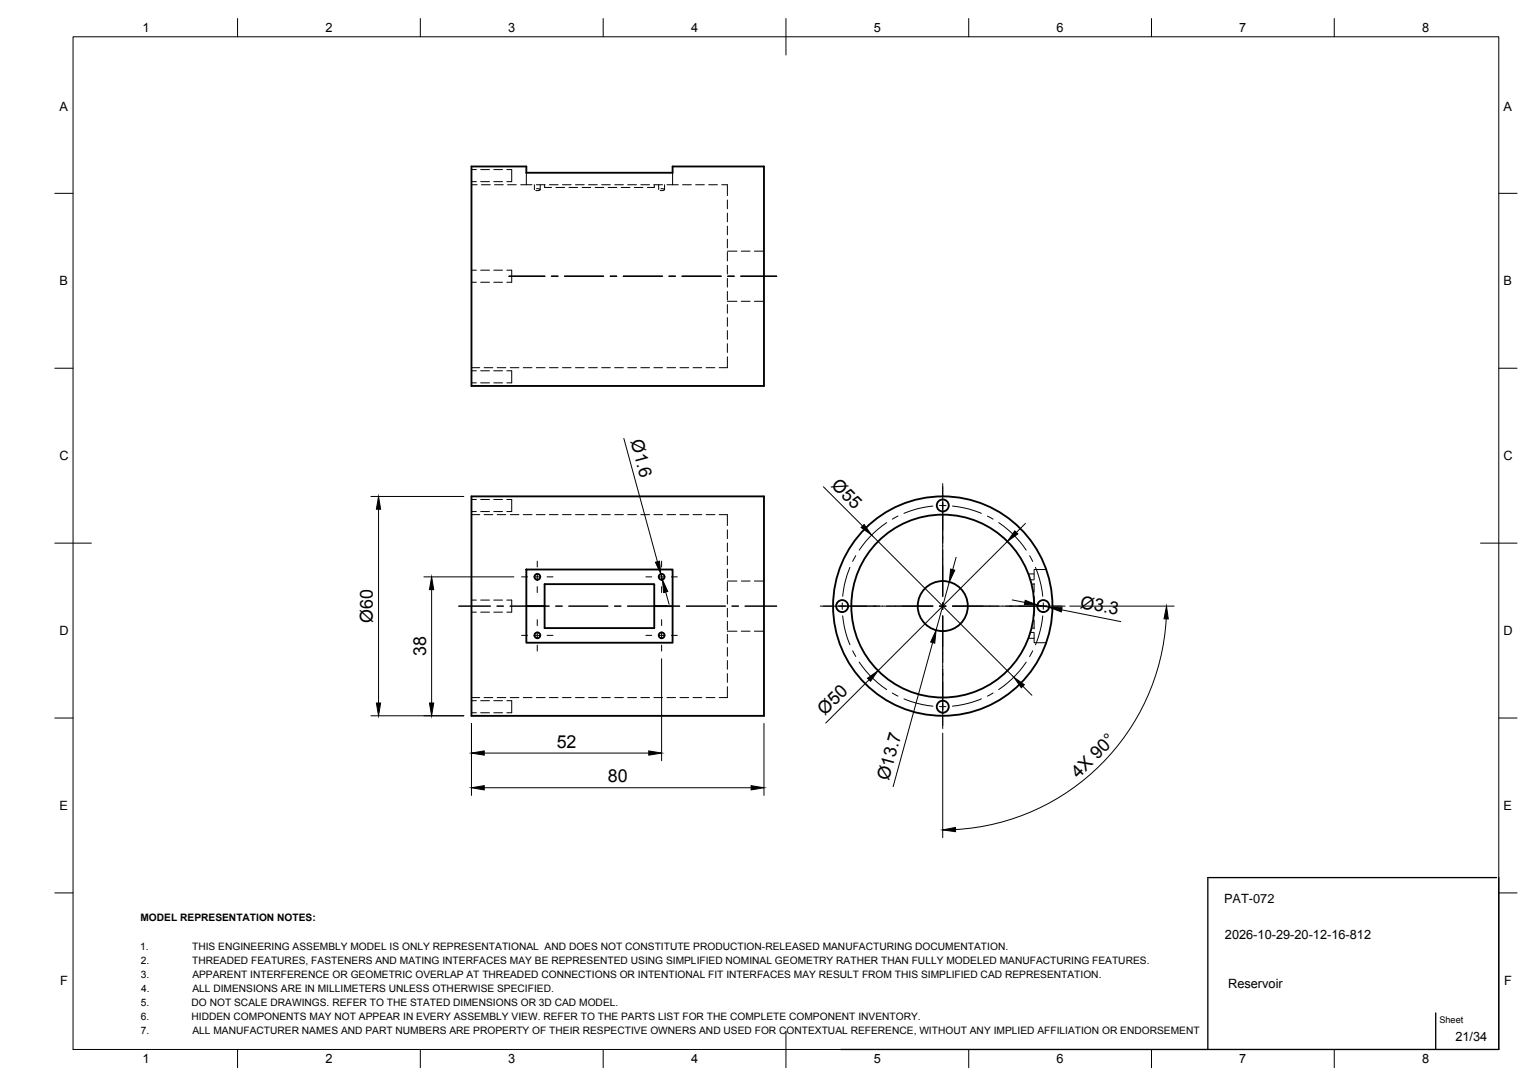
ISO-10303-21;
HEADER;
/* Generated by software containing ST-Developer
 * from STEP Tools, Inc. (www.steptools.com) 
 */

FILE_DESCRIPTION(
/* description */ ('PAT-072'),
/* implementation_level */ '2;1');

FILE_NAME(
/* name */ 'Reservoir.step',
/* time_stamp */ '2026-10-29T20:11:56-07:00',
/* author */ (''),
/* organization */ (''),
/* preprocessor_version */ 'ST-DEVELOPER v20.2',
/* originating_system */ 'Autodesk Translation Framework v15.17.0.0',
/* authorisation */ '');

FILE_SCHEMA (('AUTOMOTIVE_DESIGN { 1 0 10303 214 3 1 1 }'));
ENDSEC;

DATA;
#10=MECHANICAL_DESIGN_GEOMETRIC_PRESENTATION_REPRESENTATION('',(#350),#11432);
#249=B_SPLINE_CURVE_WITH_KNOTS('',3,(#10252,#10253,#10254,#10255,#10256,
#10257,#10258,#10259,#10260,#10261,#10262,#10263,#10264,#10265,#10266,#10267,
#10268,#10269,#10270,#10271,#10272,#10273,#10274,#10275,#10276,#10277,#10278,
#10279,#10280,#10281,#10282,#10283,#10284,#10285),.UNSPECIFIED.,.T.,.F.,
(4,2,2,2,2,2,2,2,2,2,2,2,2,2,2,2,4),(0.,0.0300404891334215,0.060080978266843,
0.0918437431465571,0.123606508026271,0.155653989866112,0.187701471705953,
0.217773943328409,0.247846414950866,0.277918886573323,0.30799135819578,
0.34003884003562,0.372086321875461,0.403849086755175,0.435611851634889,
0.465652340768311,0.495692829901732),.UNSPECIFIED.);
#250=B_SPLINE_CURVE_WITH_KNOTS('',3,(#10291,#10292,#10293,#10294,#10295,
#10296,#10297,#10298,#10299,#10300,#10301,#10302,#10303,#10304,#10305,#10306,
#10307,#10308,#10309,#10310,#10311,#10312,#10313,#10314,#10315,#10316,#10317,
#10318,#10319,#10320,#10321,#10322,#10323,#10324),.UNSPECIFIED.,.T.,.F.,
(4,2,2,2,2,2,2,2,2,2,2,2,2,2,2,2,4),(0.,0.0300724716224568,0.0601449432449135,
0.0921924250847542,0.124239906924595,0.156002671804309,0.187765436684023,
0.217805925817445,0.247846414950866,0.277886904084288,0.307927393217709,
0.339690158097423,0.371452922977137,0.403500404816978,0.435547886656819,
0.465620358279276,0.495692829901732),.UNSPECIFIED.);
#251=B_SPLINE_CURVE_WITH_KNOTS('',3,(#10330,#10331,#10332,#10333,#10334,
#10335,#10336,#10337,#10338,#10339,#10340,#10341,#10342,#10343,#10344,#10345,
#10346,#10347,#10348,#10349,#10350,#10351,#10352,#10353,#10354,#10355,#10356,
#10357,#10358,#10359,#10360,#10361,#10362,#10363),.UNSPECIFIED.,.T.,.F.,
(4,2,2,2,2,2,2,2,2,2,2,2,2,2,2,2,4),(0.,0.0300724716224568,0.0601449432449135,
0.0921924250847542,0.124239906924595,0.156002671804309,0.187765436684023,
0.217805925817445,0.247846414950866,0.277886904084288,0.307927393217709,
0.339690158097423,0.371452922977137,0.403500404816978,0.435547886656819,
0.465620358279276,0.495692829901732),.UNSPECIFIED.);
#252=B_SPLINE_CURVE_WITH_KNOTS('',3,(#10369,#10370,#10371,#10372,#10373,
#10374,#10375,#10376,#10377,#10378,#10379,#10380,#10381,#10382,#10383,#10384,
#10385,#10386,#10387,#10388,#10389,#10390,#10391,#10392,#10393,#10394,#10395,
#10396,#10397,#10398,#10399,#10400,#10401,#10402),.UNSPECIFIED.,.T.,.F.,
(4,2,2,2,2,2,2,2,2,2,2,2,2,2,2,2,4),(0.,0.0300404891334215,0.060080978266843,
0.0918437431465571,0.123606508026271,0.155653989866112,0.187701471705953,
0.217773943328409,0.247846414950866,0.277918886573323,0.30799135819578,
0.34003884003562,0.372086321875461,0.403849086755175,0.435611851634889,
0.465652340768311,0.495692829901732),.UNSPECIFIED.);
#278=SHAPE_REPRESENTATION_RELATIONSHIP('SRR','None',#11582,#314);
#314=ADVANCED_BREP_SHAPE_REPRESENTATION('',(#386),#11413);
#350=STYLED_ITEM('',(#11812),#386);
#386=MANIFOLD_SOLID_BREP('Body1',#6085);
#484=FACE_BOUND('',#1432,.T.);
#485=FACE_BOUND('',#1433,.T.);
#486=FACE_BOUND('',#1439,.T.);
#487=FACE_BOUND('',#1440,.T.);
#488=FACE_BOUND('',#1443,.T.);
#489=FACE_BOUND('',#1444,.T.);
#490=FACE_BOUND('',#1445,.T.);
#491=FACE_BOUND('',#1446,.T.);
#492=FACE_BOUND('',#1448,.T.);
#493=FACE_BOUND('',#1450,.T.);
#494=FACE_BOUND('',#1452,.T.);
#495=FACE_BOUND('',#1453,.T.);
#496=FACE_BOUND('',#1454,.T.);
#497=FACE_BOUND('',#1455,.T.);
#498=FACE_BOUND('',#1456,.T.);
#499=FACE_BOUND('',#1458,.T.);
#657=PLANE('',#6836);
#658=PLANE('',#6840);
#659=PLANE('',#6844);
#660=PLANE('',#6848);
#661=PLANE('',#6857);
#662=PLANE('',#6858);
#663=PLANE('',#6860);
#664=PLANE('',#6862);
#665=PLANE('',#6864);
#666=PLANE('',#6865);
#667=PLANE('',#6867);
#668=PLANE('',#6868);
#669=PLANE('',#6869);
#670=PLANE('',#6871);
#671=PLANE('',#6872);
#672=PLANE('',#6874);
#673=PLANE('',#6881);
#674=PLANE('',#6885);
#675=PLANE('',#6886);
#959=FACE_OUTER_BOUND('',#1413,.T.);
#960=FACE_OUTER_BOUND('',#1414,.T.);
#961=FACE_OUTER_BOUND('',#1415,.T.);
#962=FACE_OUTER_BOUND('',#1416,.T.);
#963=FACE_OUTER_BOUND('',#1417,.T.);
#964=FACE_OUTER_BOUND('',#1418,.T.);
#965=FACE_OUTER_BOUND('',#1419,.T.);
#966=FACE_OUTER_BOUND('',#1420,.T.);
#967=FACE_OUTER_BOUND('',#1421,.T.);
#968=FACE_OUTER_BOUND('',#1422,.T.);
#969=FACE_OUTER_BOUND('',#1423,.T.);
#970=FACE_OUTER_BOUND('',#1424,.T.);
#971=FACE_OUTER_BOUND('',#1425,.T.);
#972=FACE_OUTER_BOUND('',#1426,.T.);
#973=FACE_OUTER_BOUND('',#1427,.T.);
#974=FACE_OUTER_BOUND('',#1428,.T.);
#975=FACE_OUTER_BOUND('',#1429,.T.);
#976=FACE_OUTER_BOUND('',#1430,.T.);
#977=FACE_OUTER_BOUND('',#1431,.T.);
#978=FACE_OUTER_BOUND('',#1434,.T.);
#979=FACE_OUTER_BOUND('',#1435,.T.);
#980=FACE_OUTER_BOUND('',#1436,.T.);
#981=FACE_OUTER_BOUND('',#1437,.T.);
#982=FACE_OUTER_BOUND('',#1438,.T.);
#983=FACE_OUTER_BOUND('',#1441,.T.);
#984=FACE_OUTER_BOUND('',#1442,.T.);
#985=FACE_OUTER_BOUND('',#1447,.T.);
#986=FACE_OUTER_BOUND('',#1449,.T.);
#987=FACE_OUTER_BOUND('',#1451,.T.);
#988=FACE_OUTER_BOUND('',#1457,.T.);
#1413=EDGE_LOOP('',(#4678,#4679,#4680,#4681));
#1414=EDGE_LOOP('',(#4682));
#1415=EDGE_LOOP('',(#4683,#4684,#4685,#4686));
#1416=EDGE_LOOP('',(#4687));
#1417=EDGE_LOOP('',(#4688,#4689,#4690,#4691));
#1418=EDGE_LOOP('',(#4692));
#1419=EDGE_LOOP('',(#4693,#4694,#4695,#4696));
#1420=EDGE_LOOP('',(#4697));
#1421=EDGE_LOOP('',(#4698,#4699,#4700,#4701));
#1422=EDGE_LOOP('',(#4702,#4703,#4704,#4705));
#1423=EDGE_LOOP('',(#4706,#4707,#4708,#4709));
#1424=EDGE_LOOP('',(#4710,#4711,#4712,#4713));
#1425=EDGE_LOOP('',(#4714,#4715,#4716,#4717));
#1426=EDGE_LOOP('',(#4718,#4719,#4720));
#1427=EDGE_LOOP('',(#4721,#4722,#4723));
#1428=EDGE_LOOP('',(#4724,#4725,#4726));
#1429=EDGE_LOOP('',(#4727,#4728,#4729,#4730));
#1430=EDGE_LOOP('',(#4731,#4732,#4733));
#1431=EDGE_LOOP('',(#4734,#4735,#4736,#4737,#4738,#4739,#4740,#4741));
#1432=EDGE_LOOP('',(#4742));
#1433=EDGE_LOOP('',(#4743));
#1434=EDGE_LOOP('',(#4744,#4745,#4746,#4747));
#1435=EDGE_LOOP('',(#4748,#4749,#4750,#4751,#4752));
#1436=EDGE_LOOP('',(#4753,#4754,#4755,#4756));
#1437=EDGE_LOOP('',(#4757,#4758,#4759,#4760,#4761));
#1438=EDGE_LOOP('',(#4762,#4763,#4764,#4765,#4766,#4767,#4768,#4769));
#1439=EDGE_LOOP('',(#4770));
#1440=EDGE_LOOP('',(#4771));
#1441=EDGE_LOOP('',(#4772,#4773,#4774,#4775));
#1442=EDGE_LOOP('',(#4776,#4777,#4778,#4779,#4780,#4781,#4782,#4783,#4784,
#4785,#4786,#4787,#4788,#4789,#4790,#4791));
#1443=EDGE_LOOP('',(#4792));
#1444=EDGE_LOOP('',(#4793));
#1445=EDGE_LOOP('',(#4794));
#1446=EDGE_LOOP('',(#4795));
#1447=EDGE_LOOP('',(#4796));
#1448=EDGE_LOOP('',(#4797));
#1449=EDGE_LOOP('',(#4798,#4799,#4800,#4801));
#1450=EDGE_LOOP('',(#4802,#4803,#4804,#4805));
#1451=EDGE_LOOP('',(#4806));
#1452=EDGE_LOOP('',(#4807));
#1453=EDGE_LOOP('',(#4808));
#1454=EDGE_LOOP('',(#4809));
#1455=EDGE_LOOP('',(#4810));
#1456=EDGE_LOOP('',(#4811));
#1457=EDGE_LOOP('',(#4812));
#1458=EDGE_LOOP('',(#4813));
#1840=LINE('',#10223,#2259);
#1841=LINE('',#10230,#2260);
#1842=LINE('',#10237,#2261);
#1843=LINE('',#10244,#2262);
#1844=LINE('',#10251,#2263);
#1845=LINE('',#10290,#2264);
#1846=LINE('',#10329,#2265);
#1847=LINE('',#10368,#2266);
#1848=LINE('',#10406,#2267);
#1849=LINE('',#10408,#2268);
#1850=LINE('',#10410,#2269);
#1851=LINE('',#10411,#2270);
#1852=LINE('',#10417,#2271);
#1853=LINE('',#10418,#2272);
#1854=LINE('',#10424,#2273);
#1855=LINE('',#10425,#2274);
#1856=LINE('',#10428,#2275);
#1857=LINE('',#10430,#2276);
#1858=LINE('',#10431,#2277);
#1859=LINE('',#10434,#2278);
#1860=LINE('',#10437,#2279);
#1861=LINE('',#10439,#2280);
#1862=LINE('',#10441,#2281);
#1863=LINE('',#10443,#2282);
#1864=LINE('',#10444,#2283);
#1865=LINE('',#10448,#2284);
#1866=LINE('',#10449,#2285);
#1867=LINE('',#10450,#2286);
#1868=LINE('',#10455,#2287);
#1869=LINE('',#10456,#2288);
#1870=LINE('',#10459,#2289);
#1871=LINE('',#10461,#2290);
#1872=LINE('',#10462,#2291);
#1873=LINE('',#10465,#2292);
#1874=LINE('',#10467,#2293);
#1875=LINE('',#10468,#2294);
#1876=LINE('',#10473,#2295);
#1877=LINE('',#10478,#2296);
#1878=LINE('',#10480,#2297);
#1879=LINE('',#10487,#2298);
#2259=VECTOR('',#8057,0.165);
#2260=VECTOR('',#8066,0.165);
#2261=VECTOR('',#8075,0.165);
#2262=VECTOR('',#8084,0.165);
#2263=VECTOR('',#8093,0.08);
#2264=VECTOR('',#8098,0.08);
#2265=VECTOR('',#8103,0.08);
#2266=VECTOR('',#8108,0.08);
#2267=VECTOR('',#8111,1.);
#2268=VECTOR('',#8112,1.);
#2269=VECTOR('',#8113,1.);
#2270=VECTOR('',#8114,1.);
#2271=VECTOR('',#8119,1.);
#2272=VECTOR('',#8120,1.);
#2273=VECTOR('',#8125,1.);
#2274=VECTOR('',#8126,1.);
#2275=VECTOR('',#8131,1.);
#2276=VECTOR('',#8134,1.);
#2277=VECTOR('',#8135,1.);
#2278=VECTOR('',#8140,1.);
#2279=VECTOR('',#8143,1.);
#2280=VECTOR('',#8144,1.);
#2281=VECTOR('',#8145,1.);
#2282=VECTOR('',#8146,1.);
#2283=VECTOR('',#8147,1.);
#2284=VECTOR('',#8150,1.);
#2285=VECTOR('',#8151,1.);
#2286=VECTOR('',#8152,1.);
#2287=VECTOR('',#8157,1.);
#2288=VECTOR('',#8158,1.);
#2289=VECTOR('',#8161,1.);
#2290=VECTOR('',#8162,1.);
#2291=VECTOR('',#8163,1.);
#2292=VECTOR('',#8168,1.);
#2293=VECTOR('',#8171,1.);
#2294=VECTOR('',#8172,1.);
#2295=VECTOR('',#8177,0.685);
#2296=VECTOR('',#8184,2.5);
#2297=VECTOR('',#8185,2.5);
#2298=VECTOR('',#8194,3.);
#2687=CIRCLE('',#6834,0.165);
#2688=CIRCLE('',#6835,0.165);
#2689=CIRCLE('',#6838,0.165);
#2690=CIRCLE('',#6839,0.165);
#2691=CIRCLE('',#6842,0.165);
#2692=CIRCLE('',#6843,0.165);
#2693=CIRCLE('',#6846,0.165);
#2694=CIRCLE('',#6847,0.165);
#2695=CIRCLE('',#6850,0.08);
#2696=CIRCLE('',#6852,0.08);
#2697=CIRCLE('',#6854,0.08);
#2698=CIRCLE('',#6856,0.08);
#2699=CIRCLE('',#6859,2.5);
#2700=CIRCLE('',#6861,2.5);
#2701=CIRCLE('',#6863,2.5);
#2702=CIRCLE('',#6866,2.5);
#2703=CIRCLE('',#6870,3.);
#2704=CIRCLE('',#6873,3.);
#2705=CIRCLE('',#6876,0.685);
#2706=CIRCLE('',#6877,0.685);
#2707=CIRCLE('',#6879,2.5);
#2708=CIRCLE('',#6880,2.5);
#2709=CIRCLE('',#6883,3.);
#2710=CIRCLE('',#6884,3.);
#3036=VERTEX_POINT('',#10220);
#3037=VERTEX_POINT('',#10222);
#3038=VERTEX_POINT('',#10227);
#3039=VERTEX_POINT('',#10229);
#3040=VERTEX_POINT('',#10234);
#3041=VERTEX_POINT('',#10236);
#3042=VERTEX_POINT('',#10241);
#3043=VERTEX_POINT('',#10243);
#3044=VERTEX_POINT('',#10248);
#3045=VERTEX_POINT('',#10250);
#3046=VERTEX_POINT('',#10287);
#3047=VERTEX_POINT('',#10289);
#3048=VERTEX_POINT('',#10326);
#3049=VERTEX_POINT('',#10328);
#3050=VERTEX_POINT('',#10365);
#3051=VERTEX_POINT('',#10367);
#3052=VERTEX_POINT('',#10404);
#3053=VERTEX_POINT('',#10405);
#3054=VERTEX_POINT('',#10407);
#3055=VERTEX_POINT('',#10409);
#3056=VERTEX_POINT('',#10413);
#3057=VERTEX_POINT('',#10414);
#3058=VERTEX_POINT('',#10416);
#3059=VERTEX_POINT('',#10420);
#3060=VERTEX_POINT('',#10421);
#3061=VERTEX_POINT('',#10423);
#3062=VERTEX_POINT('',#10436);
#3063=VERTEX_POINT('',#10438);
#3064=VERTEX_POINT('',#10440);
#3065=VERTEX_POINT('',#10442);
#3066=VERTEX_POINT('',#10446);
#3067=VERTEX_POINT('',#10447);
#3068=VERTEX_POINT('',#10452);
#3069=VERTEX_POINT('',#10454);
#3070=VERTEX_POINT('',#10458);
#3071=VERTEX_POINT('',#10460);
#3072=VERTEX_POINT('',#10470);
#3073=VERTEX_POINT('',#10472);
#3074=VERTEX_POINT('',#10476);
#3075=VERTEX_POINT('',#10479);
#3076=VERTEX_POINT('',#10484);
#3077=VERTEX_POINT('',#10486);
#3628=EDGE_CURVE('',#3036,#3036,#2687,.T.);
#3629=EDGE_CURVE('',#3036,#3037,#1840,.T.);
#3630=EDGE_CURVE('',#3037,#3037,#2688,.T.);
#3631=EDGE_CURVE('',#3038,#3038,#2689,.T.);
#3632=EDGE_CURVE('',#3038,#3039,#1841,.T.);
#3633=EDGE_CURVE('',#3039,#3039,#2690,.T.);
#3634=EDGE_CURVE('',#3040,#3040,#2691,.T.);
#3635=EDGE_CURVE('',#3040,#3041,#1842,.T.);
#3636=EDGE_CURVE('',#3041,#3041,#2692,.T.);
#3637=EDGE_CURVE('',#3042,#3042,#2693,.T.);
#3638=EDGE_CURVE('',#3042,#3043,#1843,.T.);
#3639=EDGE_CURVE('',#3043,#3043,#2694,.T.);
#3640=EDGE_CURVE('',#3044,#3044,#2695,.T.);
#3641=EDGE_CURVE('',#3044,#3045,#1844,.T.);
#3642=EDGE_CURVE('',#3045,#3045,#249,.T.);
#3643=EDGE_CURVE('',#3046,#3046,#2696,.T.);
#3644=EDGE_CURVE('',#3046,#3047,#1845,.T.);
#3645=EDGE_CURVE('',#3047,#3047,#250,.T.);
#3646=EDGE_CURVE('',#3048,#3048,#2697,.T.);
#3647=EDGE_CURVE('',#3048,#3049,#1846,.T.);
#3648=EDGE_CURVE('',#3049,#3049,#251,.T.);
#3649=EDGE_CURVE('',#3050,#3050,#2698,.T.);
#3650=EDGE_CURVE('',#3050,#3051,#1847,.T.);
#3651=EDGE_CURVE('',#3051,#3051,#252,.T.);
#3652=EDGE_CURVE('',#3052,#3053,#1848,.T.);
#3653=EDGE_CURVE('',#3054,#3052,#1849,.T.);
#3654=EDGE_CURVE('',#3055,#3054,#1850,.T.);
#3655=EDGE_CURVE('',#3055,#3053,#1851,.T.);
#3656=EDGE_CURVE('',#3056,#3057,#2699,.T.);
#3657=EDGE_CURVE('',#3058,#3056,#1852,.T.);
#3658=EDGE_CURVE('',#3057,#3058,#1853,.T.);
#3659=EDGE_CURVE('',#3059,#3060,#2700,.T.);
#3660=EDGE_CURVE('',#3061,#3059,#1854,.T.);
#3661=EDGE_CURVE('',#3061,#3060,#1855,.T.);
#3662=EDGE_CURVE('',#3053,#3059,#2701,.T.);
#3663=EDGE_CURVE('',#3059,#3055,#1856,.T.);
#3664=EDGE_CURVE('',#3060,#3056,#1857,.T.);
#3665=EDGE_CURVE('',#3058,#3061,#1858,.T.);
#3666=EDGE_CURVE('',#3057,#3052,#2702,.T.);
#3667=EDGE_CURVE('',#3054,#3057,#1859,.T.);
#3668=EDGE_CURVE('',#3059,#3062,#1860,.T.);
#3669=EDGE_CURVE('',#3063,#3062,#1861,.T.);
#3670=EDGE_CURVE('',#3064,#3063,#1862,.T.);
#3671=EDGE_CURVE('',#3065,#3064,#1863,.T.);
#3672=EDGE_CURVE('',#3065,#3057,#1864,.T.);
#3673=EDGE_CURVE('',#3066,#3067,#1865,.T.);
#3674=EDGE_CURVE('',#3066,#3064,#1866,.T.);
#3675=EDGE_CURVE('',#3067,#3063,#1867,.T.);
#3676=EDGE_CURVE('',#3067,#3068,#2703,.T.);
#3677=EDGE_CURVE('',#3062,#3069,#1868,.T.);
#3678=EDGE_CURVE('',#3068,#3069,#1869,.T.);
#3679=EDGE_CURVE('',#3068,#3070,#1870,.T.);
#3680=EDGE_CURVE('',#3069,#3071,#1871,.T.);
#3681=EDGE_CURVE('',#3070,#3071,#1872,.T.);
#3682=EDGE_CURVE('',#3070,#3066,#2704,.T.);
#3683=EDGE_CURVE('',#3071,#3065,#1873,.T.);
#3684=EDGE_CURVE('',#3065,#3057,#1874,.T.);
#3685=EDGE_CURVE('',#3059,#3062,#1875,.T.);
#3686=EDGE_CURVE('',#3072,#3072,#2705,.T.);
#3687=EDGE_CURVE('',#3072,#3073,#1876,.T.);
#3688=EDGE_CURVE('',#3073,#3073,#2706,.T.);
#3689=EDGE_CURVE('',#3074,#3074,#2707,.T.);
#3690=EDGE_CURVE('',#3074,#3062,#1877,.T.);
#3691=EDGE_CURVE('',#3065,#3075,#1878,.T.);
#3692=EDGE_CURVE('',#3075,#3075,#2708,.T.);
#3693=EDGE_CURVE('',#3076,#3076,#2709,.T.);
#3694=EDGE_CURVE('',#3076,#3077,#1879,.T.);
#3695=EDGE_CURVE('',#3077,#3077,#2710,.T.);
#4678=ORIENTED_EDGE('',*,*,#3628,.F.);
#4679=ORIENTED_EDGE('',*,*,#3629,.T.);
#4680=ORIENTED_EDGE('',*,*,#3630,.F.);
#4681=ORIENTED_EDGE('',*,*,#3629,.F.);
#4682=ORIENTED_EDGE('',*,*,#3628,.T.);
#4683=ORIENTED_EDGE('',*,*,#3631,.F.);
#4684=ORIENTED_EDGE('',*,*,#3632,.T.);
#4685=ORIENTED_EDGE('',*,*,#3633,.F.);
#4686=ORIENTED_EDGE('',*,*,#3632,.F.);
#4687=ORIENTED_EDGE('',*,*,#3631,.T.);
#4688=ORIENTED_EDGE('',*,*,#3634,.F.);
#4689=ORIENTED_EDGE('',*,*,#3635,.T.);
#4690=ORIENTED_EDGE('',*,*,#3636,.F.);
#4691=ORIENTED_EDGE('',*,*,#3635,.F.);
#4692=ORIENTED_EDGE('',*,*,#3634,.T.);
#4693=ORIENTED_EDGE('',*,*,#3637,.F.);
#4694=ORIENTED_EDGE('',*,*,#3638,.T.);
#4695=ORIENTED_EDGE('',*,*,#3639,.F.);
#4696=ORIENTED_EDGE('',*,*,#3638,.F.);
#4697=ORIENTED_EDGE('',*,*,#3637,.T.);
#4698=ORIENTED_EDGE('',*,*,#3640,.F.);
#4699=ORIENTED_EDGE('',*,*,#3641,.T.);
#4700=ORIENTED_EDGE('',*,*,#3642,.F.);
#4701=ORIENTED_EDGE('',*,*,#3641,.F.);
#4702=ORIENTED_EDGE('',*,*,#3643,.F.);
#4703=ORIENTED_EDGE('',*,*,#3644,.T.);
#4704=ORIENTED_EDGE('',*,*,#3645,.F.);
#4705=ORIENTED_EDGE('',*,*,#3644,.F.);
#4706=ORIENTED_EDGE('',*,*,#3646,.F.);
#4707=ORIENTED_EDGE('',*,*,#3647,.T.);
#4708=ORIENTED_EDGE('',*,*,#3648,.F.);
#4709=ORIENTED_EDGE('',*,*,#3647,.F.);
#4710=ORIENTED_EDGE('',*,*,#3649,.F.);
#4711=ORIENTED_EDGE('',*,*,#3650,.T.);
#4712=ORIENTED_EDGE('',*,*,#3651,.F.);
#4713=ORIENTED_EDGE('',*,*,#3650,.F.);
#4714=ORIENTED_EDGE('',*,*,#3652,.F.);
#4715=ORIENTED_EDGE('',*,*,#3653,.F.);
#4716=ORIENTED_EDGE('',*,*,#3654,.F.);
#4717=ORIENTED_EDGE('',*,*,#3655,.T.);
#4718=ORIENTED_EDGE('',*,*,#3656,.F.);
#4719=ORIENTED_EDGE('',*,*,#3657,.F.);
#4720=ORIENTED_EDGE('',*,*,#3658,.F.);
#4721=ORIENTED_EDGE('',*,*,#3659,.F.);
#4722=ORIENTED_EDGE('',*,*,#3660,.F.);
#4723=ORIENTED_EDGE('',*,*,#3661,.T.);
#4724=ORIENTED_EDGE('',*,*,#3662,.F.);
#4725=ORIENTED_EDGE('',*,*,#3655,.F.);
#4726=ORIENTED_EDGE('',*,*,#3663,.F.);
#4727=ORIENTED_EDGE('',*,*,#3664,.F.);
#4728=ORIENTED_EDGE('',*,*,#3661,.F.);
#4729=ORIENTED_EDGE('',*,*,#3665,.F.);
#4730=ORIENTED_EDGE('',*,*,#3657,.T.);
#4731=ORIENTED_EDGE('',*,*,#3666,.F.);
#4732=ORIENTED_EDGE('',*,*,#3667,.F.);
#4733=ORIENTED_EDGE('',*,*,#3653,.T.);
#4734=ORIENTED_EDGE('',*,*,#3658,.T.);
#4735=ORIENTED_EDGE('',*,*,#3665,.T.);
#4736=ORIENTED_EDGE('',*,*,#3660,.T.);
#4737=ORIENTED_EDGE('',*,*,#3668,.T.);
#4738=ORIENTED_EDGE('',*,*,#3669,.F.);
#4739=ORIENTED_EDGE('',*,*,#3670,.F.);
#4740=ORIENTED_EDGE('',*,*,#3671,.F.);
#4741=ORIENTED_EDGE('',*,*,#3672,.T.);
#4742=ORIENTED_EDGE('',*,*,#3640,.T.);
#4743=ORIENTED_EDGE('',*,*,#3649,.T.);
#4744=ORIENTED_EDGE('',*,*,#3673,.F.);
#4745=ORIENTED_EDGE('',*,*,#3674,.T.);
#4746=ORIENTED_EDGE('',*,*,#3670,.T.);
#4747=ORIENTED_EDGE('',*,*,#3675,.F.);
#4748=ORIENTED_EDGE('',*,*,#3676,.F.);
#4749=ORIENTED_EDGE('',*,*,#3675,.T.);
#4750=ORIENTED_EDGE('',*,*,#3669,.T.);
#4751=ORIENTED_EDGE('',*,*,#3677,.T.);
#4752=ORIENTED_EDGE('',*,*,#3678,.F.);
#4753=ORIENTED_EDGE('',*,*,#3679,.F.);
#4754=ORIENTED_EDGE('',*,*,#3678,.T.);
#4755=ORIENTED_EDGE('',*,*,#3680,.T.);
#4756=ORIENTED_EDGE('',*,*,#3681,.F.);
#4757=ORIENTED_EDGE('',*,*,#3682,.F.);
#4758=ORIENTED_EDGE('',*,*,#3681,.T.);
#4759=ORIENTED_EDGE('',*,*,#3683,.T.);
#4760=ORIENTED_EDGE('',*,*,#3671,.T.);
#4761=ORIENTED_EDGE('',*,*,#3674,.F.);
#4762=ORIENTED_EDGE('',*,*,#3667,.T.);
#4763=ORIENTED_EDGE('',*,*,#3684,.F.);
#4764=ORIENTED_EDGE('',*,*,#3683,.F.);
#4765=ORIENTED_EDGE('',*,*,#3680,.F.);
#4766=ORIENTED_EDGE('',*,*,#3677,.F.);
#4767=ORIENTED_EDGE('',*,*,#3685,.F.);
#4768=ORIENTED_EDGE('',*,*,#3663,.T.);
#4769=ORIENTED_EDGE('',*,*,#3654,.T.);
#4770=ORIENTED_EDGE('',*,*,#3643,.T.);
#4771=ORIENTED_EDGE('',*,*,#3646,.T.);
#4772=ORIENTED_EDGE('',*,*,#3686,.F.);
#4773=ORIENTED_EDGE('',*,*,#3687,.T.);
#4774=ORIENTED_EDGE('',*,*,#3688,.F.);
#4775=ORIENTED_EDGE('',*,*,#3687,.F.);
#4776=ORIENTED_EDGE('',*,*,#3689,.F.);
#4777=ORIENTED_EDGE('',*,*,#3690,.T.);
#4778=ORIENTED_EDGE('',*,*,#3668,.F.);
#4779=ORIENTED_EDGE('',*,*,#3659,.T.);
#4780=ORIENTED_EDGE('',*,*,#3664,.T.);
#4781=ORIENTED_EDGE('',*,*,#3656,.T.);
#4782=ORIENTED_EDGE('',*,*,#3672,.F.);
#4783=ORIENTED_EDGE('',*,*,#3691,.T.);
#4784=ORIENTED_EDGE('',*,*,#3692,.F.);
#4785=ORIENTED_EDGE('',*,*,#3691,.F.);
#4786=ORIENTED_EDGE('',*,*,#3684,.T.);
#4787=ORIENTED_EDGE('',*,*,#3666,.T.);
#4788=ORIENTED_EDGE('',*,*,#3652,.T.);
#4789=ORIENTED_EDGE('',*,*,#3662,.T.);
#4790=ORIENTED_EDGE('',*,*,#3685,.T.);
#4791=ORIENTED_EDGE('',*,*,#3690,.F.);
#4792=ORIENTED_EDGE('',*,*,#3642,.T.);
#4793=ORIENTED_EDGE('',*,*,#3645,.T.);
#4794=ORIENTED_EDGE('',*,*,#3648,.T.);
#4795=ORIENTED_EDGE('',*,*,#3651,.T.);
#4796=ORIENTED_EDGE('',*,*,#3689,.T.);
#4797=ORIENTED_EDGE('',*,*,#3688,.T.);
#4798=ORIENTED_EDGE('',*,*,#3693,.F.);
#4799=ORIENTED_EDGE('',*,*,#3694,.T.);
#4800=ORIENTED_EDGE('',*,*,#3695,.T.);
#4801=ORIENTED_EDGE('',*,*,#3694,.F.);
#4802=ORIENTED_EDGE('',*,*,#3679,.T.);
#4803=ORIENTED_EDGE('',*,*,#3682,.T.);
#4804=ORIENTED_EDGE('',*,*,#3673,.T.);
#4805=ORIENTED_EDGE('',*,*,#3676,.T.);
#4806=ORIENTED_EDGE('',*,*,#3693,.T.);
#4807=ORIENTED_EDGE('',*,*,#3692,.T.);
#4808=ORIENTED_EDGE('',*,*,#3639,.T.);
#4809=ORIENTED_EDGE('',*,*,#3636,.T.);
#4810=ORIENTED_EDGE('',*,*,#3633,.T.);
#4811=ORIENTED_EDGE('',*,*,#3630,.T.);
#4812=ORIENTED_EDGE('',*,*,#3695,.F.);
#4813=ORIENTED_EDGE('',*,*,#3686,.T.);
#5634=CYLINDRICAL_SURFACE('',#6833,0.165);
#5635=CYLINDRICAL_SURFACE('',#6837,0.165);
#5636=CYLINDRICAL_SURFACE('',#6841,0.165);
#5637=CYLINDRICAL_SURFACE('',#6845,0.165);
#5638=CYLINDRICAL_SURFACE('',#6849,0.08);
#5639=CYLINDRICAL_SURFACE('',#6851,0.08);
#5640=CYLINDRICAL_SURFACE('',#6853,0.08);
#5641=CYLINDRICAL_SURFACE('',#6855,0.08);
#5642=CYLINDRICAL_SURFACE('',#6875,0.685);
#5643=CYLINDRICAL_SURFACE('',#6878,2.5);
#5644=CYLINDRICAL_SURFACE('',#6882,3.);
#5858=ADVANCED_FACE('',(#959),#5634,.F.);
#5859=ADVANCED_FACE('',(#960),#657,.T.);
#5860=ADVANCED_FACE('',(#961),#5635,.F.);
#5861=ADVANCED_FACE('',(#962),#658,.T.);
#5862=ADVANCED_FACE('',(#963),#5636,.F.);
#5863=ADVANCED_FACE('',(#964),#659,.T.);
#5864=ADVANCED_FACE('',(#965),#5637,.F.);
#5865=ADVANCED_FACE('',(#966),#660,.T.);
#5866=ADVANCED_FACE('',(#967),#5638,.F.);
#5867=ADVANCED_FACE('',(#968),#5639,.F.);
#5868=ADVANCED_FACE('',(#969),#5640,.F.);
#5869=ADVANCED_FACE('',(#970),#5641,.F.);
#5870=ADVANCED_FACE('',(#971),#661,.F.);
#5871=ADVANCED_FACE('',(#972),#662,.F.);
#5872=ADVANCED_FACE('',(#973),#663,.F.);
#5873=ADVANCED_FACE('',(#974),#664,.F.);
#5874=ADVANCED_FACE('',(#975),#665,.F.);
#5875=ADVANCED_FACE('',(#976),#666,.F.);
#5876=ADVANCED_FACE('',(#977,#484,#485),#667,.F.);
#5877=ADVANCED_FACE('',(#978),#668,.F.);
#5878=ADVANCED_FACE('',(#979),#669,.F.);
#5879=ADVANCED_FACE('',(#980),#670,.F.);
#5880=ADVANCED_FACE('',(#981),#671,.F.);
#5881=ADVANCED_FACE('',(#982,#486,#487),#672,.F.);
#5882=ADVANCED_FACE('',(#983),#5642,.F.);
#5883=ADVANCED_FACE('',(#984,#488,#489,#490,#491),#5643,.F.);
#5884=ADVANCED_FACE('',(#985,#492),#673,.T.);
#5885=ADVANCED_FACE('',(#986,#493),#5644,.T.);
#5886=ADVANCED_FACE('',(#987,#494,#495,#496,#497,#498),#674,.T.);
#5887=ADVANCED_FACE('',(#988,#499),#675,.F.);
#6085=CLOSED_SHELL('',(#5858,#5859,#5860,#5861,#5862,#5863,#5864,#5865,
#5866,#5867,#5868,#5869,#5870,#5871,#5872,#5873,#5874,#5875,#5876,#5877,
#5878,#5879,#5880,#5881,#5882,#5883,#5884,#5885,#5886,#5887));
#6832=AXIS2_PLACEMENT_3D('',#10218,#8051,#8052);
#6833=AXIS2_PLACEMENT_3D('',#10219,#8053,#8054);
#6834=AXIS2_PLACEMENT_3D('',#10221,#8055,#8056);
#6835=AXIS2_PLACEMENT_3D('',#10224,#8058,#8059);
#6836=AXIS2_PLACEMENT_3D('',#10225,#8060,#8061);
#6837=AXIS2_PLACEMENT_3D('',#10226,#8062,#8063);
#6838=AXIS2_PLACEMENT_3D('',#10228,#8064,#8065);
#6839=AXIS2_PLACEMENT_3D('',#10231,#8067,#8068);
#6840=AXIS2_PLACEMENT_3D('',#10232,#8069,#8070);
#6841=AXIS2_PLACEMENT_3D('',#10233,#8071,#8072);
#6842=AXIS2_PLACEMENT_3D('',#10235,#8073,#8074);
#6843=AXIS2_PLACEMENT_3D('',#10238,#8076,#8077);
#6844=AXIS2_PLACEMENT_3D('',#10239,#8078,#8079);
#6845=AXIS2_PLACEMENT_3D('',#10240,#8080,#8081);
#6846=AXIS2_PLACEMENT_3D('',#10242,#8082,#8083);
#6847=AXIS2_PLACEMENT_3D('',#10245,#8085,#8086);
#6848=AXIS2_PLACEMENT_3D('',#10246,#8087,#8088);
#6849=AXIS2_PLACEMENT_3D('',#10247,#8089,#8090);
#6850=AXIS2_PLACEMENT_3D('',#10249,#8091,#8092);
#6851=AXIS2_PLACEMENT_3D('',#10286,#8094,#8095);
#6852=AXIS2_PLACEMENT_3D('',#10288,#8096,#8097);
#6853=AXIS2_PLACEMENT_3D('',#10325,#8099,#8100);
#6854=AXIS2_PLACEMENT_3D('',#10327,#8101,#8102);
#6855=AXIS2_PLACEMENT_3D('',#10364,#8104,#8105);
#6856=AXIS2_PLACEMENT_3D('',#10366,#8106,#8107);
#6857=AXIS2_PLACEMENT_3D('',#10403,#8109,#8110);
#6858=AXIS2_PLACEMENT_3D('',#10412,#8115,#8116);
#6859=AXIS2_PLACEMENT_3D('',#10415,#8117,#8118);
#6860=AXIS2_PLACEMENT_3D('',#10419,#8121,#8122);
#6861=AXIS2_PLACEMENT_3D('',#10422,#8123,#8124);
#6862=AXIS2_PLACEMENT_3D('',#10426,#8127,#8128);
#6863=AXIS2_PLACEMENT_3D('',#10427,#8129,#8130);
#6864=AXIS2_PLACEMENT_3D('',#10429,#8132,#8133);
#6865=AXIS2_PLACEMENT_3D('',#10432,#8136,#8137);
#6866=AXIS2_PLACEMENT_3D('',#10433,#8138,#8139);
#6867=AXIS2_PLACEMENT_3D('',#10435,#8141,#8142);
#6868=AXIS2_PLACEMENT_3D('',#10445,#8148,#8149);
#6869=AXIS2_PLACEMENT_3D('',#10451,#8153,#8154);
#6870=AXIS2_PLACEMENT_3D('',#10453,#8155,#8156);
#6871=AXIS2_PLACEMENT_3D('',#10457,#8159,#8160);
#6872=AXIS2_PLACEMENT_3D('',#10463,#8164,#8165);
#6873=AXIS2_PLACEMENT_3D('',#10464,#8166,#8167);
#6874=AXIS2_PLACEMENT_3D('',#10466,#8169,#8170);
#6875=AXIS2_PLACEMENT_3D('',#10469,#8173,#8174);
#6876=AXIS2_PLACEMENT_3D('',#10471,#8175,#8176);
#6877=AXIS2_PLACEMENT_3D('',#10474,#8178,#8179);
#6878=AXIS2_PLACEMENT_3D('',#10475,#8180,#8181);
#6879=AXIS2_PLACEMENT_3D('',#10477,#8182,#8183);
#6880=AXIS2_PLACEMENT_3D('',#10481,#8186,#8187);
#6881=AXIS2_PLACEMENT_3D('',#10482,#8188,#8189);
#6882=AXIS2_PLACEMENT_3D('',#10483,#8190,#8191);
#6883=AXIS2_PLACEMENT_3D('',#10485,#8192,#8193);
#6884=AXIS2_PLACEMENT_3D('',#10488,#8195,#8196);
#6885=AXIS2_PLACEMENT_3D('',#10489,#8197,#8198);
#6886=AXIS2_PLACEMENT_3D('',#10490,#8199,#8200);
#8051=DIRECTION('axis',(0.,0.,1.));
#8052=DIRECTION('refdir',(1.,0.,0.));
#8053=DIRECTION('center_axis',(0.,0.,1.));
#8054=DIRECTION('ref_axis',(1.,0.,0.));
#8055=DIRECTION('center_axis',(0.,0.,1.));
#8056=DIRECTION('ref_axis',(1.,0.,0.));
#8057=DIRECTION('',(0.,0.,1.));
#8058=DIRECTION('center_axis',(0.,0.,-1.));
#8059=DIRECTION('ref_axis',(1.,0.,0.));
#8060=DIRECTION('center_axis',(0.,0.,1.));
#8061=DIRECTION('ref_axis',(1.,0.,0.));
#8062=DIRECTION('center_axis',(0.,0.,1.));
#8063=DIRECTION('ref_axis',(1.,0.,0.));
#8064=DIRECTION('center_axis',(0.,0.,1.));
#8065=DIRECTION('ref_axis',(1.,0.,0.));
#8066=DIRECTION('',(0.,0.,1.));
#8067=DIRECTION('center_axis',(0.,0.,-1.));
#8068=DIRECTION('ref_axis',(1.,0.,0.));
#8069=DIRECTION('center_axis',(0.,0.,1.));
#8070=DIRECTION('ref_axis',(1.,0.,0.));
#8071=DIRECTION('center_axis',(0.,0.,1.));
#8072=DIRECTION('ref_axis',(1.,0.,0.));
#8073=DIRECTION('center_axis',(0.,0.,1.));
#8074=DIRECTION('ref_axis',(1.,0.,0.));
#8075=DIRECTION('',(0.,0.,1.));
#8076=DIRECTION('center_axis',(0.,0.,-1.));
#8077=DIRECTION('ref_axis',(1.,0.,0.));
#8078=DIRECTION('center_axis',(0.,0.,1.));
#8079=DIRECTION('ref_axis',(1.,0.,0.));
#8080=DIRECTION('center_axis',(0.,0.,1.));
#8081=DIRECTION('ref_axis',(1.,0.,0.));
#8082=DIRECTION('center_axis',(0.,0.,1.));
#8083=DIRECTION('ref_axis',(1.,0.,0.));
#8084=DIRECTION('',(0.,0.,1.));
#8085=DIRECTION('center_axis',(0.,0.,-1.));
#8086=DIRECTION('ref_axis',(1.,0.,0.));
#8087=DIRECTION('center_axis',(0.,0.,1.));
#8088=DIRECTION('ref_axis',(1.,0.,0.));
#8089=DIRECTION('center_axis',(0.,1.,0.));
#8090=DIRECTION('ref_axis',(1.,0.,0.));
#8091=DIRECTION('center_axis',(0.,1.,0.));
#8092=DIRECTION('ref_axis',(1.,0.,0.));
#8093=DIRECTION('',(0.,1.,0.));
#8094=DIRECTION('center_axis',(0.,1.,0.));
#8095=DIRECTION('ref_axis',(1.,0.,0.));
#8096=DIRECTION('center_axis',(0.,1.,0.));
#8097=DIRECTION('ref_axis',(1.,0.,0.));
#8098=DIRECTION('',(0.,1.,0.));
#8099=DIRECTION('center_axis',(0.,1.,0.));
#8100=DIRECTION('ref_axis',(1.,0.,0.));
#8101=DIRECTION('center_axis',(0.,1.,0.));
#8102=DIRECTION('ref_axis',(1.,0.,0.));
#8103=DIRECTION('',(0.,1.,0.));
#8104=DIRECTION('center_axis',(0.,1.,0.));
#8105=DIRECTION('ref_axis',(1.,0.,0.));
#8106=DIRECTION('center_axis',(0.,1.,0.));
#8107=DIRECTION('ref_axis',(1.,0.,0.));
#8108=DIRECTION('',(0.,1.,0.));
#8109=DIRECTION('center_axis',(-1.,0.,0.));
#8110=DIRECTION('ref_axis',(0.,0.,1.));
#8111=DIRECTION('',(0.,0.,-1.));
#8112=DIRECTION('',(0.,1.,0.));
#8113=DIRECTION('',(0.,0.,1.));
#8114=DIRECTION('',(0.,1.,0.));
#8115=DIRECTION('center_axis',(0.,0.,1.));
#8116=DIRECTION('ref_axis',(1.,0.,0.));
#8117=DIRECTION('center_axis',(0.,0.,-1.));
#8118=DIRECTION('ref_axis',(1.,0.,0.));
#8119=DIRECTION('',(0.,1.,0.));
#8120=DIRECTION('',(1.,0.,0.));
#8121=DIRECTION('center_axis',(0.,0.,-1.));
#8122=DIRECTION('ref_axis',(-1.,0.,0.));
#8123=DIRECTION('center_axis',(0.,0.,1.));
#8124=DIRECTION('ref_axis',(1.,0.,0.));
#8125=DIRECTION('',(-1.,0.,0.));
#8126=DIRECTION('',(0.,1.,0.));
#8127=DIRECTION('center_axis',(0.,0.,-1.));
#8128=DIRECTION('ref_axis',(-1.,0.,0.));
#8129=DIRECTION('center_axis',(0.,0.,1.));
#8130=DIRECTION('ref_axis',(1.,0.,0.));
#8131=DIRECTION('',(-1.,0.,0.));
#8132=DIRECTION('center_axis',(1.,0.,0.));
#8133=DIRECTION('ref_axis',(0.,0.,-1.));
#8134=DIRECTION('',(0.,0.,1.));
#8135=DIRECTION('',(0.,0.,-1.));
#8136=DIRECTION('center_axis',(0.,0.,1.));
#8137=DIRECTION('ref_axis',(1.,0.,0.));
#8138=DIRECTION('center_axis',(0.,0.,-1.));
#8139=DIRECTION('ref_axis',(1.,0.,0.));
#8140=DIRECTION('',(1.,0.,0.));
#8141=DIRECTION('center_axis',(0.,1.,0.));
#8142=DIRECTION('ref_axis',(0.,0.,1.));
#8143=DIRECTION('',(0.,0.,-1.));
#8144=DIRECTION('',(-1.,0.,0.));
#8145=DIRECTION('',(0.,0.,-1.));
#8146=DIRECTION('',(1.,0.,0.));
#8147=DIRECTION('',(0.,0.,-1.));
#8148=DIRECTION('center_axis',(1.,0.,0.));
#8149=DIRECTION('ref_axis',(0.,0.,-1.));
#8150=DIRECTION('',(0.,0.,-1.));
#8151=DIRECTION('',(0.,1.,0.));
#8152=DIRECTION('',(0.,1.,0.));
#8153=DIRECTION('center_axis',(0.,0.,-1.));
#8154=DIRECTION('ref_axis',(-1.,0.,0.));
#8155=DIRECTION('center_axis',(0.,0.,-1.));
#8156=DIRECTION('ref_axis',(1.,0.,0.));
#8157=DIRECTION('',(-1.,0.,0.));
#8158=DIRECTION('',(0.,1.,0.));
#8159=DIRECTION('center_axis',(-1.,0.,0.));
#8160=DIRECTION('ref_axis',(0.,0.,1.));
#8161=DIRECTION('',(0.,0.,1.));
#8162=DIRECTION('',(0.,0.,1.));
#8163=DIRECTION('',(0.,1.,0.));
#8164=DIRECTION('center_axis',(0.,0.,1.));
#8165=DIRECTION('ref_axis',(1.,0.,0.));
#8166=DIRECTION('center_axis',(0.,0.,1.));
#8167=DIRECTION('ref_axis',(1.,0.,0.));
#8168=DIRECTION('',(1.,0.,0.));
#8169=DIRECTION('center_axis',(0.,1.,0.));
#8170=DIRECTION('ref_axis',(0.,0.,1.));
#8171=DIRECTION('',(0.,0.,-1.));
#8172=DIRECTION('',(0.,0.,-1.));
#8173=DIRECTION('center_axis',(0.,0.,1.));
#8174=DIRECTION('ref_axis',(1.,0.,0.));
#8175=DIRECTION('center_axis',(0.,0.,1.));
#8176=DIRECTION('ref_axis',(1.,0.,0.));
#8177=DIRECTION('',(0.,0.,1.));
#8178=DIRECTION('center_axis',(0.,0.,-1.));
#8179=DIRECTION('ref_axis',(1.,0.,0.));
#8180=DIRECTION('center_axis',(0.,0.,1.));
#8181=DIRECTION('ref_axis',(6.12323399573677E-17,1.,0.));
#8182=DIRECTION('center_axis',(0.,0.,1.));
#8183=DIRECTION('ref_axis',(1.,0.,0.));
#8184=DIRECTION('',(0.,0.,1.));
#8185=DIRECTION('',(0.,0.,1.));
#8186=DIRECTION('center_axis',(0.,0.,-1.));
#8187=DIRECTION('ref_axis',(1.,0.,0.));
#8188=DIRECTION('center_axis',(0.,0.,1.));
#8189=DIRECTION('ref_axis',(1.,0.,0.));
#8190=DIRECTION('center_axis',(0.,0.,1.));
#8191=DIRECTION('ref_axis',(1.,0.,0.));
#8192=DIRECTION('center_axis',(0.,0.,1.));
#8193=DIRECTION('ref_axis',(1.,0.,0.));
#8194=DIRECTION('',(0.,0.,-1.));
#8195=DIRECTION('center_axis',(0.,0.,1.));
#8196=DIRECTION('ref_axis',(1.,0.,0.));
#8197=DIRECTION('center_axis',(0.,0.,1.));
#8198=DIRECTION('ref_axis',(1.,0.,0.));
#8199=DIRECTION('center_axis',(0.,0.,1.));
#8200=DIRECTION('ref_axis',(1.,0.,0.));
#10218=CARTESIAN_POINT('',(0.,0.,0.));
#10219=CARTESIAN_POINT('Origin',(-2.75,3.36777869765522E-16,13.9));
#10220=CARTESIAN_POINT('',(-2.915,3.16571197579591E-16,13.9));
#10221=CARTESIAN_POINT('Origin',(-2.75,3.36777869765522E-16,13.9));
#10222=CARTESIAN_POINT('',(-2.915,3.56984541951453E-16,15.));
#10223=CARTESIAN_POINT('',(-2.915,3.16571197579591E-16,13.9));
#10224=CARTESIAN_POINT('Origin',(-2.75,3.36777869765522E-16,15.));
#10225=CARTESIAN_POINT('Origin',(-2.75,3.33066907387547E-16,13.9));
#10226=CARTESIAN_POINT('Origin',(1.68388934882761E-16,2.75,13.9));
#10227=CARTESIAN_POINT('',(-0.165,2.75,13.9));
#10228=CARTESIAN_POINT('Origin',(1.68388934882761E-16,2.75,13.9));
#10229=CARTESIAN_POINT('',(-0.165,2.75,15.));
#10230=CARTESIAN_POINT('',(-0.165,2.75,13.9));
#10231=CARTESIAN_POINT('Origin',(1.68388934882761E-16,2.75,15.));
#10232=CARTESIAN_POINT('Origin',(1.66533453693773E-16,2.75,13.9));
#10233=CARTESIAN_POINT('Origin',(2.75,0.,13.9));
#10234=CARTESIAN_POINT('',(2.585,-2.02066721859313E-17,13.9));
#10235=CARTESIAN_POINT('Origin',(2.75,0.,13.9));
#10236=CARTESIAN_POINT('',(2.585,2.02066721859313E-17,15.));
#10237=CARTESIAN_POINT('',(2.585,-2.02066721859313E-17,13.9));
#10238=CARTESIAN_POINT('Origin',(2.75,0.,15.));
#10239=CARTESIAN_POINT('Origin',(2.75,0.,13.9));
#10240=CARTESIAN_POINT('Origin',(-5.05166804648283E-16,-2.75,13.9));
#10241=CARTESIAN_POINT('',(-0.165,-2.75,13.9));
#10242=CARTESIAN_POINT('Origin',(-5.05166804648283E-16,-2.75,13.9));
#10243=CARTESIAN_POINT('',(-0.165,-2.75,15.));
#10244=CARTESIAN_POINT('',(-0.165,-2.75,13.9));
#10245=CARTESIAN_POINT('Origin',(-5.05166804648283E-16,-2.75,15.));
#10246=CARTESIAN_POINT('Origin',(-4.9960036108132E-16,-2.75,13.9));
#10247=CARTESIAN_POINT('Origin',(0.8,-2.6,9.8));
#10248=CARTESIAN_POINT('',(0.72,-2.5,9.8));
#10249=CARTESIAN_POINT('Origin',(0.8,-2.5,9.8));
#10250=CARTESIAN_POINT('',(0.72,-2.39407602218476,9.8));
#10251=CARTESIAN_POINT('',(0.72,-2.6,9.8));
#10252=CARTESIAN_POINT('Ctrl Pts',(0.72,-2.39407602218476,9.8));
#10253=CARTESIAN_POINT('Ctrl Pts',(0.72,-2.39407602218476,9.78998650362219));
#10254=CARTESIAN_POINT('Ctrl Pts',(0.721997829419093,-2.39347795314806,
9.77933670746212));
#10255=CARTESIAN_POINT('Ctrl Pts',(0.730021672239828,-2.39104285533446,
9.75982110231822));
#10256=CARTESIAN_POINT('Ctrl Pts',(0.736044837862985,-2.38920269063634,
9.75095451399836));
#10257=CARTESIAN_POINT('Ctrl Pts',(0.750142086204369,-2.3848153859957,9.73658705643568));
#10258=CARTESIAN_POINT('Ctrl Pts',(0.759292738749644,-2.38192864200441,
9.73029163224123));
#10259=CARTESIAN_POINT('Ctrl Pts',(0.779207514547847,-2.37548840620605,
9.72199993483929));
#10260=CARTESIAN_POINT('Ctrl Pts',(0.789969133117306,-2.37193188471924,
9.72));
#10261=CARTESIAN_POINT('Ctrl Pts',(0.810120782163592,-2.36512545840249,
9.72));
#10262=CARTESIAN_POINT('Ctrl Pts',(0.820924889571242,-2.36139662819874,
9.72203247425743));
#10263=CARTESIAN_POINT('Ctrl Pts',(0.840861824541038,-2.35437106294126,
9.73037890165789));
#10264=CARTESIAN_POINT('Ctrl Pts',(0.849995310916174,-2.35107789272744,
9.73669428134057));
#10265=CARTESIAN_POINT('Ctrl Pts',(0.864015479756631,-2.34596024152528,
9.75104732679704));
#10266=CARTESIAN_POINT('Ctrl Pts',(0.87000322488351,-2.34373901948205,9.75987236006433));
#10267=CARTESIAN_POINT('Ctrl Pts',(0.877997733074498,-2.34075590003467,
9.77933523544702));
#10268=CARTESIAN_POINT('Ctrl Pts',(0.88,-2.34,9.78997584279251));
#10269=CARTESIAN_POINT('Ctrl Pts',(0.88,-2.34,9.81002415720749));
#10270=CARTESIAN_POINT('Ctrl Pts',(0.877997733074498,-2.34075590003467,
9.82066476455298));
#10271=CARTESIAN_POINT('Ctrl Pts',(0.87000322488351,-2.34373901948205,9.84012763993567));
#10272=CARTESIAN_POINT('Ctrl Pts',(0.864015479756631,-2.34596024152528,
9.84895267320296));
#10273=CARTESIAN_POINT('Ctrl Pts',(0.849995310916174,-2.35107789272744,
9.86330571865944));
#10274=CARTESIAN_POINT('Ctrl Pts',(0.840861824541038,-2.35437106294126,
9.86962109834211));
#10275=CARTESIAN_POINT('Ctrl Pts',(0.820924889571242,-2.36139662819874,
9.87796752574257));
#10276=CARTESIAN_POINT('Ctrl Pts',(0.810120782163592,-2.36512545840249,
9.88));
#10277=CARTESIAN_POINT('Ctrl Pts',(0.789969133117306,-2.37193188471924,
9.88));
#10278=CARTESIAN_POINT('Ctrl Pts',(0.779207514547847,-2.37548840620605,
9.87800006516071));
#10279=CARTESIAN_POINT('Ctrl Pts',(0.759292738749644,-2.38192864200441,
9.86970836775877));
#10280=CARTESIAN_POINT('Ctrl Pts',(0.750142086204369,-2.3848153859957,9.86341294356432));
#10281=CARTESIAN_POINT('Ctrl Pts',(0.736044837862985,-2.38920269063634,
9.84904548600165));
#10282=CARTESIAN_POINT('Ctrl Pts',(0.730021672239828,-2.39104285533446,
9.84017889768178));
#10283=CARTESIAN_POINT('Ctrl Pts',(0.721997829419093,-2.39347795314806,
9.82066329253788));
#10284=CARTESIAN_POINT('Ctrl Pts',(0.72,-2.39407602218476,9.81001349637781));
#10285=CARTESIAN_POINT('Ctrl Pts',(0.72,-2.39407602218476,9.8));
#10286=CARTESIAN_POINT('Origin',(-0.8,-2.6,13.2));
#10287=CARTESIAN_POINT('',(-0.88,-2.5,13.2));
#10288=CARTESIAN_POINT('Origin',(-0.8,-2.5,13.2));
#10289=CARTESIAN_POINT('',(-0.88,-2.34,13.2));
#10290=CARTESIAN_POINT('',(-0.88,-2.6,13.2));
#10291=CARTESIAN_POINT('Ctrl Pts',(-0.88,-2.34,13.2));
#10292=CARTESIAN_POINT('Ctrl Pts',(-0.88,-2.34,13.1899758427925));
#10293=CARTESIAN_POINT('Ctrl Pts',(-0.877997733074498,-2.34075590003467,
13.179335235447));
#10294=CARTESIAN_POINT('Ctrl Pts',(-0.87000322488351,-2.34373901948205,
13.1598723600643));
#10295=CARTESIAN_POINT('Ctrl Pts',(-0.864015479756631,-2.34596024152528,
13.151047326797));
#10296=CARTESIAN_POINT('Ctrl Pts',(-0.849995310916174,-2.35107789272744,
13.1366942813406));
#10297=CARTESIAN_POINT('Ctrl Pts',(-0.840861824541038,-2.35437106294126,
13.1303789016579));
#10298=CARTESIAN_POINT('Ctrl Pts',(-0.820924889571242,-2.36139662819874,
13.1220324742574));
#10299=CARTESIAN_POINT('Ctrl Pts',(-0.810120782163592,-2.36512545840249,
13.12));
#10300=CARTESIAN_POINT('Ctrl Pts',(-0.789969133117306,-2.37193188471924,
13.12));
#10301=CARTESIAN_POINT('Ctrl Pts',(-0.779207514547847,-2.37548840620605,
13.1219999348393));
#10302=CARTESIAN_POINT('Ctrl Pts',(-0.759292738749644,-2.38192864200441,
13.1302916322412));
#10303=CARTESIAN_POINT('Ctrl Pts',(-0.750142086204369,-2.3848153859957,
13.1365870564357));
#10304=CARTESIAN_POINT('Ctrl Pts',(-0.736044837862985,-2.38920269063634,
13.1509545139984));
#10305=CARTESIAN_POINT('Ctrl Pts',(-0.730021672239828,-2.39104285533446,
13.1598211023182));
#10306=CARTESIAN_POINT('Ctrl Pts',(-0.721997829419093,-2.39347795314806,
13.1793367074621));
#10307=CARTESIAN_POINT('Ctrl Pts',(-0.72,-2.39407602218476,13.1899865036222));
#10308=CARTESIAN_POINT('Ctrl Pts',(-0.72,-2.39407602218476,13.2100134963778));
#10309=CARTESIAN_POINT('Ctrl Pts',(-0.721997829419093,-2.39347795314806,
13.2206632925379));
#10310=CARTESIAN_POINT('Ctrl Pts',(-0.730021672239828,-2.39104285533446,
13.2401788976818));
#10311=CARTESIAN_POINT('Ctrl Pts',(-0.736044837862985,-2.38920269063634,
13.2490454860016));
#10312=CARTESIAN_POINT('Ctrl Pts',(-0.750142086204369,-2.3848153859957,
13.2634129435643));
#10313=CARTESIAN_POINT('Ctrl Pts',(-0.759292738749644,-2.38192864200441,
13.2697083677588));
#10314=CARTESIAN_POINT('Ctrl Pts',(-0.779207514547847,-2.37548840620605,
13.2780000651607));
#10315=CARTESIAN_POINT('Ctrl Pts',(-0.789969133117306,-2.37193188471924,
13.28));
#10316=CARTESIAN_POINT('Ctrl Pts',(-0.810120782163592,-2.36512545840249,
13.28));
#10317=CARTESIAN_POINT('Ctrl Pts',(-0.820924889571242,-2.36139662819874,
13.2779675257426));
#10318=CARTESIAN_POINT('Ctrl Pts',(-0.840861824541038,-2.35437106294126,
13.2696210983421));
#10319=CARTESIAN_POINT('Ctrl Pts',(-0.849995310916174,-2.35107789272744,
13.2633057186594));
#10320=CARTESIAN_POINT('Ctrl Pts',(-0.864015479756631,-2.34596024152528,
13.248952673203));
#10321=CARTESIAN_POINT('Ctrl Pts',(-0.87000322488351,-2.34373901948205,
13.2401276399357));
#10322=CARTESIAN_POINT('Ctrl Pts',(-0.877997733074498,-2.34075590003467,
13.220664764553));
#10323=CARTESIAN_POINT('Ctrl Pts',(-0.88,-2.34,13.2100241572075));
#10324=CARTESIAN_POINT('Ctrl Pts',(-0.88,-2.34,13.2));
#10325=CARTESIAN_POINT('Origin',(-0.8,-2.6,9.8));
#10326=CARTESIAN_POINT('',(-0.88,-2.5,9.8));
#10327=CARTESIAN_POINT('Origin',(-0.8,-2.5,9.8));
#10328=CARTESIAN_POINT('',(-0.88,-2.34,9.8));
#10329=CARTESIAN_POINT('',(-0.88,-2.6,9.8));
#10330=CARTESIAN_POINT('Ctrl Pts',(-0.88,-2.34,9.8));
#10331=CARTESIAN_POINT('Ctrl Pts',(-0.88,-2.34,9.78997584279251));
#10332=CARTESIAN_POINT('Ctrl Pts',(-0.877997733074498,-2.34075590003467,
9.77933523544702));
#10333=CARTESIAN_POINT('Ctrl Pts',(-0.87000322488351,-2.34373901948205,
9.75987236006433));
#10334=CARTESIAN_POINT('Ctrl Pts',(-0.864015479756631,-2.34596024152528,
9.75104732679704));
#10335=CARTESIAN_POINT('Ctrl Pts',(-0.849995310916174,-2.35107789272744,
9.73669428134057));
#10336=CARTESIAN_POINT('Ctrl Pts',(-0.840861824541038,-2.35437106294126,
9.73037890165789));
#10337=CARTESIAN_POINT('Ctrl Pts',(-0.820924889571242,-2.36139662819874,
9.72203247425743));
#10338=CARTESIAN_POINT('Ctrl Pts',(-0.810120782163592,-2.36512545840249,
9.72));
#10339=CARTESIAN_POINT('Ctrl Pts',(-0.789969133117306,-2.37193188471924,
9.72));
#10340=CARTESIAN_POINT('Ctrl Pts',(-0.779207514547847,-2.37548840620605,
9.72199993483929));
#10341=CARTESIAN_POINT('Ctrl Pts',(-0.759292738749644,-2.38192864200441,
9.73029163224123));
#10342=CARTESIAN_POINT('Ctrl Pts',(-0.750142086204369,-2.3848153859957,
9.73658705643568));
#10343=CARTESIAN_POINT('Ctrl Pts',(-0.736044837862985,-2.38920269063634,
9.75095451399836));
#10344=CARTESIAN_POINT('Ctrl Pts',(-0.730021672239828,-2.39104285533446,
9.75982110231822));
#10345=CARTESIAN_POINT('Ctrl Pts',(-0.721997829419093,-2.39347795314806,
9.77933670746212));
#10346=CARTESIAN_POINT('Ctrl Pts',(-0.72,-2.39407602218476,9.78998650362219));
#10347=CARTESIAN_POINT('Ctrl Pts',(-0.72,-2.39407602218476,9.81001349637781));
#10348=CARTESIAN_POINT('Ctrl Pts',(-0.721997829419093,-2.39347795314806,
9.82066329253788));
#10349=CARTESIAN_POINT('Ctrl Pts',(-0.730021672239828,-2.39104285533446,
9.84017889768178));
#10350=CARTESIAN_POINT('Ctrl Pts',(-0.736044837862985,-2.38920269063634,
9.84904548600165));
#10351=CARTESIAN_POINT('Ctrl Pts',(-0.750142086204369,-2.3848153859957,
9.86341294356432));
#10352=CARTESIAN_POINT('Ctrl Pts',(-0.759292738749644,-2.38192864200441,
9.86970836775877));
#10353=CARTESIAN_POINT('Ctrl Pts',(-0.779207514547847,-2.37548840620605,
9.87800006516071));
#10354=CARTESIAN_POINT('Ctrl Pts',(-0.789969133117306,-2.37193188471924,
9.88));
#10355=CARTESIAN_POINT('Ctrl Pts',(-0.810120782163592,-2.36512545840249,
9.88));
#10356=CARTESIAN_POINT('Ctrl Pts',(-0.820924889571242,-2.36139662819874,
9.87796752574257));
#10357=CARTESIAN_POINT('Ctrl Pts',(-0.840861824541038,-2.35437106294126,
9.86962109834211));
#10358=CARTESIAN_POINT('Ctrl Pts',(-0.849995310916174,-2.35107789272744,
9.86330571865944));
#10359=CARTESIAN_POINT('Ctrl Pts',(-0.864015479756631,-2.34596024152528,
9.84895267320296));
#10360=CARTESIAN_POINT('Ctrl Pts',(-0.87000322488351,-2.34373901948205,
9.84012763993567));
#10361=CARTESIAN_POINT('Ctrl Pts',(-0.877997733074498,-2.34075590003467,
9.82066476455298));
#10362=CARTESIAN_POINT('Ctrl Pts',(-0.88,-2.34,9.81002415720748));
#10363=CARTESIAN_POINT('Ctrl Pts',(-0.88,-2.34,9.8));
#10364=CARTESIAN_POINT('Origin',(0.8,-2.6,13.2));
#10365=CARTESIAN_POINT('',(0.72,-2.5,13.2));
#10366=CARTESIAN_POINT('Origin',(0.8,-2.5,13.2));
#10367=CARTESIAN_POINT('',(0.72,-2.39407602218476,13.2));
#10368=CARTESIAN_POINT('',(0.72,-2.6,13.2));
#10369=CARTESIAN_POINT('Ctrl Pts',(0.72,-2.39407602218476,13.2));
#10370=CARTESIAN_POINT('Ctrl Pts',(0.72,-2.39407602218476,13.1899865036222));
#10371=CARTESIAN_POINT('Ctrl Pts',(0.721997829419093,-2.39347795314806,
13.1793367074621));
#10372=CARTESIAN_POINT('Ctrl Pts',(0.730021672239828,-2.39104285533446,
13.1598211023182));
#10373=CARTESIAN_POINT('Ctrl Pts',(0.736044837862985,-2.38920269063634,
13.1509545139984));
#10374=CARTESIAN_POINT('Ctrl Pts',(0.750142086204369,-2.3848153859957,13.1365870564357));
#10375=CARTESIAN_POINT('Ctrl Pts',(0.759292738749644,-2.38192864200441,
13.1302916322412));
#10376=CARTESIAN_POINT('Ctrl Pts',(0.779207514547847,-2.37548840620605,
13.1219999348393));
#10377=CARTESIAN_POINT('Ctrl Pts',(0.789969133117306,-2.37193188471924,
13.12));
#10378=CARTESIAN_POINT('Ctrl Pts',(0.810120782163592,-2.36512545840249,
13.12));
#10379=CARTESIAN_POINT('Ctrl Pts',(0.820924889571242,-2.36139662819874,
13.1220324742574));
#10380=CARTESIAN_POINT('Ctrl Pts',(0.840861824541038,-2.35437106294126,
13.1303789016579));
#10381=CARTESIAN_POINT('Ctrl Pts',(0.849995310916174,-2.35107789272744,
13.1366942813406));
#10382=CARTESIAN_POINT('Ctrl Pts',(0.864015479756631,-2.34596024152528,
13.151047326797));
#10383=CARTESIAN_POINT('Ctrl Pts',(0.87000322488351,-2.34373901948205,13.1598723600643));
#10384=CARTESIAN_POINT('Ctrl Pts',(0.877997733074498,-2.34075590003467,
13.179335235447));
#10385=CARTESIAN_POINT('Ctrl Pts',(0.88,-2.34,13.1899758427925));
#10386=CARTESIAN_POINT('Ctrl Pts',(0.88,-2.34,13.2100241572075));
#10387=CARTESIAN_POINT('Ctrl Pts',(0.877997733074498,-2.34075590003467,
13.220664764553));
#10388=CARTESIAN_POINT('Ctrl Pts',(0.87000322488351,-2.34373901948205,13.2401276399357));
#10389=CARTESIAN_POINT('Ctrl Pts',(0.864015479756631,-2.34596024152528,
13.248952673203));
#10390=CARTESIAN_POINT('Ctrl Pts',(0.849995310916174,-2.35107789272744,
13.2633057186594));
#10391=CARTESIAN_POINT('Ctrl Pts',(0.840861824541038,-2.35437106294126,
13.2696210983421));
#10392=CARTESIAN_POINT('Ctrl Pts',(0.820924889571242,-2.36139662819874,
13.2779675257426));
#10393=CARTESIAN_POINT('Ctrl Pts',(0.810120782163592,-2.36512545840249,
13.28));
#10394=CARTESIAN_POINT('Ctrl Pts',(0.789969133117306,-2.37193188471924,
13.28));
#10395=CARTESIAN_POINT('Ctrl Pts',(0.779207514547847,-2.37548840620605,
13.2780000651607));
#10396=CARTESIAN_POINT('Ctrl Pts',(0.759292738749644,-2.38192864200441,
13.2697083677588));
#10397=CARTESIAN_POINT('Ctrl Pts',(0.750142086204369,-2.3848153859957,13.2634129435643));
#10398=CARTESIAN_POINT('Ctrl Pts',(0.736044837862985,-2.38920269063634,
13.2490454860016));
#10399=CARTESIAN_POINT('Ctrl Pts',(0.730021672239828,-2.39104285533446,
13.2401788976818));
#10400=CARTESIAN_POINT('Ctrl Pts',(0.721997829419093,-2.39347795314806,
13.2206632925379));
#10401=CARTESIAN_POINT('Ctrl Pts',(0.72,-2.39407602218476,13.2100134963778));
#10402=CARTESIAN_POINT('Ctrl Pts',(0.72,-2.39407602218476,13.2));
#10403=CARTESIAN_POINT('Origin',(-0.6,-3.1,10.));
#10404=CARTESIAN_POINT('',(-0.6,-2.42693221990232,13.));
#10405=CARTESIAN_POINT('',(-0.6,-2.42693221990232,10.));
#10406=CARTESIAN_POINT('',(-0.6,-2.42693221990232,8.));
#10407=CARTESIAN_POINT('',(-0.6,-2.5,13.));
#10408=CARTESIAN_POINT('',(-0.6,-3.1,13.));
#10409=CARTESIAN_POINT('',(-0.6,-2.5,10.));
#10410=CARTESIAN_POINT('',(-0.6,-2.5,10.75));
#10411=CARTESIAN_POINT('',(-0.6,-3.1,10.));
#10412=CARTESIAN_POINT('Origin',(-0.6,-3.1,13.));
#10413=CARTESIAN_POINT('',(0.6,-2.42693221990232,13.));
#10414=CARTESIAN_POINT('',(0.,-2.5,13.));
#10415=CARTESIAN_POINT('Origin',(0.,0.,13.));
#10416=CARTESIAN_POINT('',(0.6,-2.5,13.));
#10417=CARTESIAN_POINT('',(0.6,-3.1,13.));
#10418=CARTESIAN_POINT('',(-0.3,-2.5,13.));
#10419=CARTESIAN_POINT('Origin',(0.6,-3.1,10.));
#10420=CARTESIAN_POINT('',(0.,-2.5,10.));
#10421=CARTESIAN_POINT('',(0.6,-2.42693221990232,10.));
#10422=CARTESIAN_POINT('Origin',(0.,0.,10.));
#10423=CARTESIAN_POINT('',(0.6,-2.5,10.));
#10424=CARTESIAN_POINT('',(0.3,-2.5,10.));
#10425=CARTESIAN_POINT('',(0.6,-3.1,10.));
#10426=CARTESIAN_POINT('Origin',(0.6,-3.1,10.));
#10427=CARTESIAN_POINT('Origin',(0.,0.,10.));
#10428=CARTESIAN_POINT('',(0.3,-2.5,10.));
#10429=CARTESIAN_POINT('Origin',(0.6,-3.1,13.));
#10430=CARTESIAN_POINT('',(0.6,-2.42693221990232,8.));
#10431=CARTESIAN_POINT('',(0.6,-2.5,12.25));
#10432=CARTESIAN_POINT('Origin',(-0.6,-3.1,13.));
#10433=CARTESIAN_POINT('Origin',(0.,0.,13.));
#10434=CARTESIAN_POINT('',(-0.3,-2.5,13.));
#10435=CARTESIAN_POINT('Origin',(0.,-2.5,11.5));
#10436=CARTESIAN_POINT('',(0.,-2.5,9.5));
#10437=CARTESIAN_POINT('',(0.,-2.5,8.));
#10438=CARTESIAN_POINT('',(1.,-2.5,9.5));
#10439=CARTESIAN_POINT('',(-1.,-2.5,9.5));
#10440=CARTESIAN_POINT('',(1.,-2.5,13.5));
#10441=CARTESIAN_POINT('',(1.,-2.5,9.5));
#10442=CARTESIAN_POINT('',(0.,-2.5,13.5));
#10443=CARTESIAN_POINT('',(1.,-2.5,13.5));
#10444=CARTESIAN_POINT('',(0.,-2.5,8.));
#10445=CARTESIAN_POINT('Origin',(1.,-3.1,13.5));
#10446=CARTESIAN_POINT('',(1.,-2.82842712474619,13.5));
#10447=CARTESIAN_POINT('',(1.,-2.82842712474619,9.5));
#10448=CARTESIAN_POINT('',(1.,-2.82842712474619,7.));
#10449=CARTESIAN_POINT('',(1.,-3.1,13.5));
#10450=CARTESIAN_POINT('',(1.,-3.1,9.5));
#10451=CARTESIAN_POINT('Origin',(1.,-3.1,9.5));
#10452=CARTESIAN_POINT('',(-1.,-2.82842712474619,9.5));
#10453=CARTESIAN_POINT('Origin',(0.,0.,9.5));
#10454=CARTESIAN_POINT('',(-1.,-2.5,9.5));
#10455=CARTESIAN_POINT('',(-1.,-2.5,9.5));
#10456=CARTESIAN_POINT('',(-1.,-3.1,9.5));
#10457=CARTESIAN_POINT('Origin',(-1.,-3.1,9.5));
#10458=CARTESIAN_POINT('',(-1.,-2.82842712474619,13.5));
#10459=CARTESIAN_POINT('',(-1.,-2.82842712474619,7.));
#10460=CARTESIAN_POINT('',(-1.,-2.5,13.5));
#10461=CARTESIAN_POINT('',(-1.,-2.5,13.5));
#10462=CARTESIAN_POINT('',(-1.,-3.1,13.5));
#10463=CARTESIAN_POINT('Origin',(-1.,-3.1,13.5));
#10464=CARTESIAN_POINT('Origin',(0.,0.,13.5));
#10465=CARTESIAN_POINT('',(1.,-2.5,13.5));
#10466=CARTESIAN_POINT('Origin',(0.,-2.5,11.5));
#10467=CARTESIAN_POINT('',(0.,-2.5,8.));
#10468=CARTESIAN_POINT('',(0.,-2.5,8.));
#10469=CARTESIAN_POINT('Origin',(0.,0.,6.9));
#10470=CARTESIAN_POINT('',(-0.685,-8.38883057415937E-17,7.));
#10471=CARTESIAN_POINT('Origin',(0.,0.,7.));
#10472=CARTESIAN_POINT('',(-0.685,8.38883057415937E-17,8.));
#10473=CARTESIAN_POINT('',(-0.685,-8.38883057415937E-17,6.9));
#10474=CARTESIAN_POINT('Origin',(0.,0.,8.));
#10475=CARTESIAN_POINT('Origin',(0.,0.,8.));
#10476=CARTESIAN_POINT('',(1.53080849893419E-16,-2.5,8.));
#10477=CARTESIAN_POINT('Origin',(0.,0.,8.));
#10478=CARTESIAN_POINT('',(1.53080849893419E-16,-2.5,8.));
#10479=CARTESIAN_POINT('',(1.53080849893419E-16,-2.5,15.));
#10480=CARTESIAN_POINT('',(1.53080849893419E-16,-2.5,8.));
#10481=CARTESIAN_POINT('Origin',(0.,0.,15.));
#10482=CARTESIAN_POINT('Origin',(0.,0.,8.));
#10483=CARTESIAN_POINT('Origin',(0.,0.,7.));
#10484=CARTESIAN_POINT('',(-3.,-3.67394039744206E-16,15.));
#10485=CARTESIAN_POINT('Origin',(0.,0.,15.));
#10486=CARTESIAN_POINT('',(-3.,-3.67394039744206E-16,7.));
#10487=CARTESIAN_POINT('',(-3.,-3.67394039744206E-16,7.));
#10488=CARTESIAN_POINT('Origin',(0.,0.,7.));
#10489=CARTESIAN_POINT('Origin',(0.,0.,15.));
#10490=CARTESIAN_POINT('Origin',(0.,0.,7.));
#11374=UNCERTAINTY_MEASURE_WITH_UNIT(LENGTH_MEASURE(0.001),#11433,
'DISTANCE_ACCURACY_VALUE',
'Maximum model space distance between geometric entities at asserted c
onnectivities');
#11393=UNCERTAINTY_MEASURE_WITH_UNIT(LENGTH_MEASURE(0.001),#11433,
'DISTANCE_ACCURACY_VALUE',
'Maximum model space distance between geometric entities at asserted c
onnectivities');
#11413=(
GEOMETRIC_REPRESENTATION_CONTEXT(3)
GLOBAL_UNCERTAINTY_ASSIGNED_CONTEXT((#11374))
GLOBAL_UNIT_ASSIGNED_CONTEXT((#11433,#11435,#11436))
REPRESENTATION_CONTEXT('','3D')
);
#11432=(
GEOMETRIC_REPRESENTATION_CONTEXT(3)
GLOBAL_UNCERTAINTY_ASSIGNED_CONTEXT((#11393))
GLOBAL_UNIT_ASSIGNED_CONTEXT((#11433,#11435,#11436))
REPRESENTATION_CONTEXT('','3D')
);
#11433=(
LENGTH_UNIT()
NAMED_UNIT(*)
SI_UNIT(.CENTI.,.METRE.)
);
#11435=(
NAMED_UNIT(*)
PLANE_ANGLE_UNIT()
SI_UNIT($,.RADIAN.)
);
#11436=(
NAMED_UNIT(*)
SI_UNIT($,.STERADIAN.)
SOLID_ANGLE_UNIT()
);
#11456=SHAPE_DEFINITION_REPRESENTATION(#11494,#11582);
#11494=PRODUCT_DEFINITION_SHAPE('',$,#11621);
#11582=SHAPE_REPRESENTATION('',(#6832),#11413);
#11601=PRODUCT_DEFINITION_CONTEXT('part definition',#11717,'design');
#11621=PRODUCT_DEFINITION('Reservoir','Reservoir',#11659,
#11601);
#11659=PRODUCT_DEFINITION_FORMATION('',$,#11738);
#11717=APPLICATION_CONTEXT(
'Core Data for Automotive Mechanical Design Process');
#11718=PRODUCT_CONTEXT('part definition',#11717,'mechanical');
#11738=PRODUCT('Reservoir','Reservoir','Reservoir',(#11718));
#11806=COLOUR_RGB('Sky Blue',0.24,0.69,0.87);
#11807=FILL_AREA_STYLE_COLOUR('',#11806);
#11808=FILL_AREA_STYLE('',(#11807));
#11809=SURFACE_STYLE_FILL_AREA(#11808);
#11810=SURFACE_SIDE_STYLE('',(#11809));
#11811=SURFACE_STYLE_USAGE(.BOTH.,#11810);
#11812=PRESENTATION_STYLE_ASSIGNMENT((#11811));
ENDSEC;
END-ISO-10303-21;
